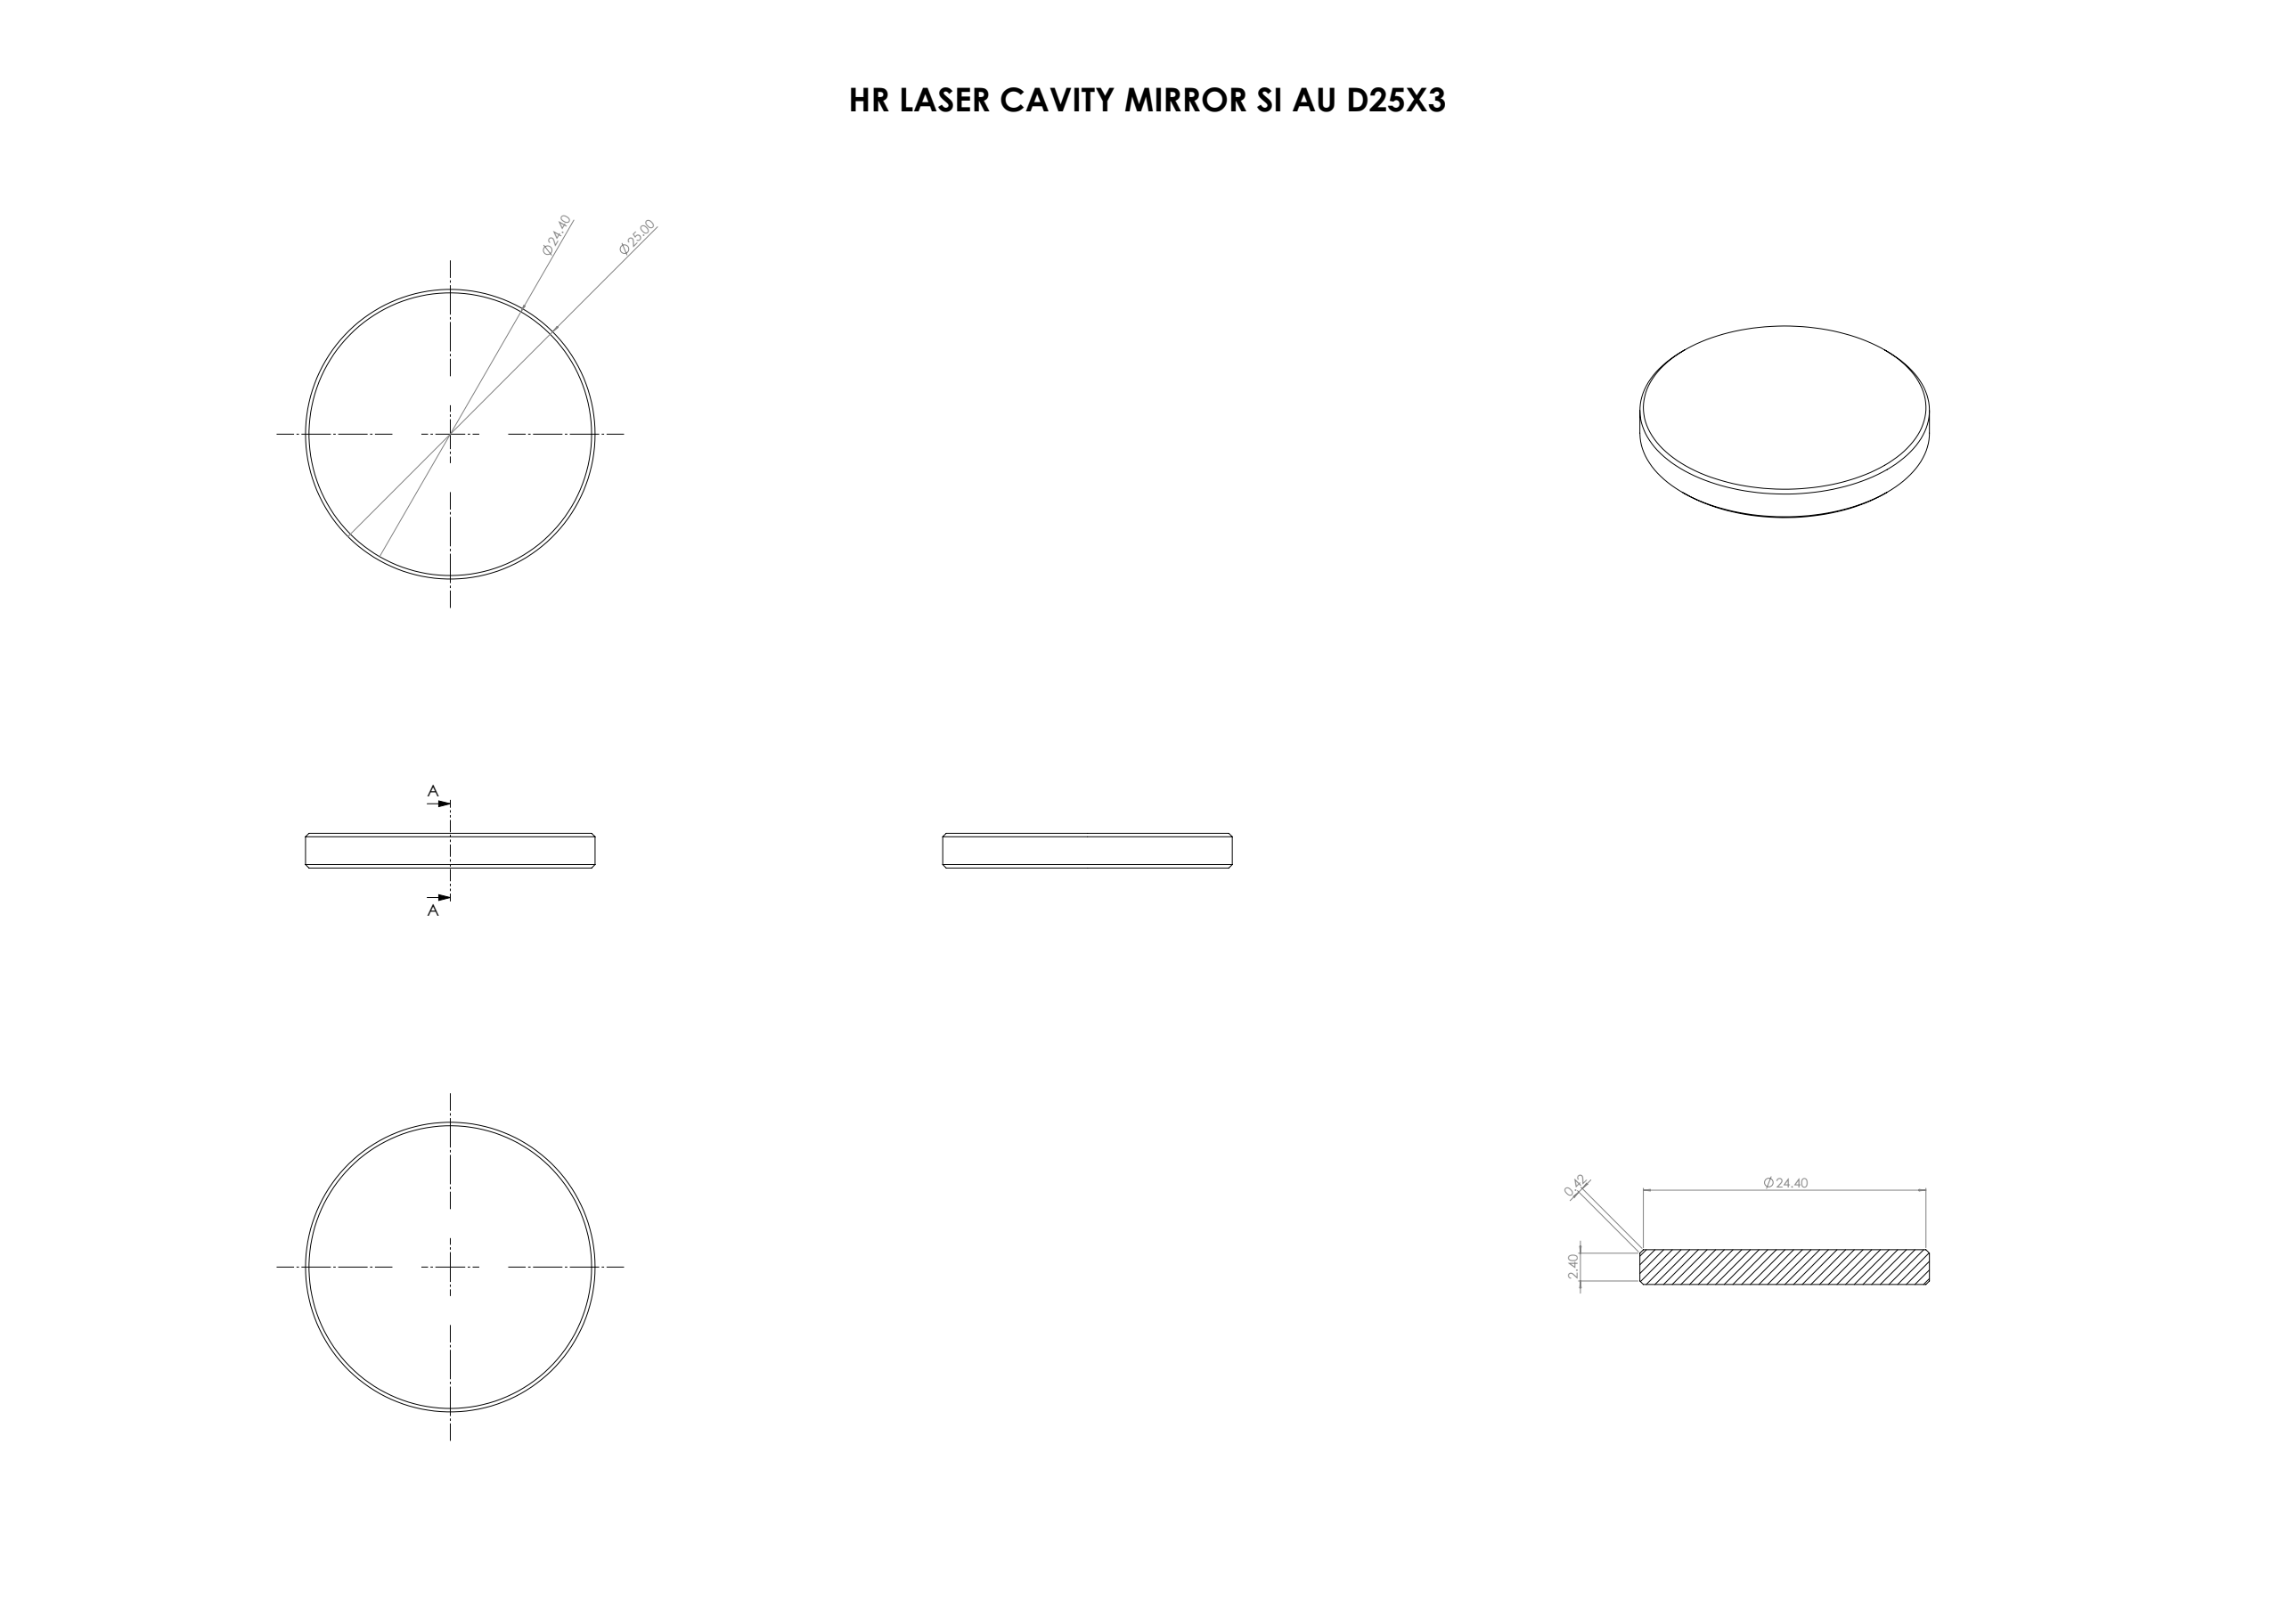
ISO-10303-21;
HEADER;
/* Generated by software containing ST-Developer
 * from STEP Tools, Inc. (www.steptools.com) 
 */

FILE_DESCRIPTION(
/* description */ (''),
/* implementation_level */ '2;1');

FILE_NAME(
/* name */ 
'06_HR_Laser_Cavity_Mirror_Si_Au_D25x3.step',
/* time_stamp */ '2026-10-20T10:06:23-07:00',
/* author */ (''),
/* organization */ (''),
/* preprocessor_version */ 'ST-DEVELOPER v20.2',
/* originating_system */ 'Autodesk Translation Framework v15.15.0.0',
/* authorisation */ '');

FILE_SCHEMA (('AUTOMOTIVE_DESIGN { 1 0 10303 214 3 1 1 }'));
ENDSEC;

DATA;
#10=MECHANICAL_DESIGN_GEOMETRIC_PRESENTATION_REPRESENTATION('',(#464),#38611);
#436=SHAPE_REPRESENTATION_RELATIONSHIP('SRR','None',#38672,#450);
#450=ADVANCED_BREP_SHAPE_REPRESENTATION('',(#478),#38601);
#464=STYLED_ITEM('',(#38871),#478);
#478=MANIFOLD_SOLID_BREP('Mirror',#16238);
#906=CYLINDRICAL_SURFACE('',#16779,1.25);
#1337=CIRCLE('',#16776,1.22);
#1338=CIRCLE('',#16778,1.25);
#1339=CIRCLE('',#16780,1.25);
#1340=CIRCLE('',#16782,1.22);
#1733=CONICAL_SURFACE('',#16777,1.235,0.785398163397449);
#1734=CONICAL_SURFACE('',#16781,1.235,0.78539816339745);
#2010=FACE_OUTER_BOUND('',#2953,.T.);
#2011=FACE_OUTER_BOUND('',#2954,.T.);
#2012=FACE_OUTER_BOUND('',#2955,.T.);
#2013=FACE_OUTER_BOUND('',#2956,.T.);
#2014=FACE_OUTER_BOUND('',#2957,.T.);
#2953=EDGE_LOOP('',(#11173));
#2954=EDGE_LOOP('',(#11174,#11175,#11176,#11177));
#2955=EDGE_LOOP('',(#11178,#11179,#11180,#11181));
#2956=EDGE_LOOP('',(#11182,#11183,#11184,#11185));
#2957=EDGE_LOOP('',(#11186));
#4081=LINE('',#23395,#5305);
#4082=LINE('',#23399,#5306);
#4083=LINE('',#23403,#5307);
#5305=VECTOR('',#18984,1.235);
#5306=VECTOR('',#18989,1.25);
#5307=VECTOR('',#18994,1.235);
#6459=VERTEX_POINT('',#23390);
#6460=VERTEX_POINT('',#23393);
#6461=VERTEX_POINT('',#23397);
#6462=VERTEX_POINT('',#23401);
#8202=EDGE_CURVE('',#6459,#6459,#1337,.T.);
#8203=EDGE_CURVE('',#6460,#6460,#1338,.T.);
#8204=EDGE_CURVE('',#6460,#6459,#4081,.T.);
#8205=EDGE_CURVE('',#6461,#6461,#1339,.T.);
#8206=EDGE_CURVE('',#6461,#6460,#4082,.T.);
#8207=EDGE_CURVE('',#6462,#6462,#1340,.T.);
#8208=EDGE_CURVE('',#6462,#6461,#4083,.T.);
#11173=ORIENTED_EDGE('',*,*,#8202,.F.);
#11174=ORIENTED_EDGE('',*,*,#8203,.F.);
#11175=ORIENTED_EDGE('',*,*,#8204,.T.);
#11176=ORIENTED_EDGE('',*,*,#8202,.T.);
#11177=ORIENTED_EDGE('',*,*,#8204,.F.);
#11178=ORIENTED_EDGE('',*,*,#8205,.F.);
#11179=ORIENTED_EDGE('',*,*,#8206,.T.);
#11180=ORIENTED_EDGE('',*,*,#8203,.T.);
#11181=ORIENTED_EDGE('',*,*,#8206,.F.);
#11182=ORIENTED_EDGE('',*,*,#8207,.F.);
#11183=ORIENTED_EDGE('',*,*,#8208,.T.);
#11184=ORIENTED_EDGE('',*,*,#8205,.T.);
#11185=ORIENTED_EDGE('',*,*,#8208,.F.);
#11186=ORIENTED_EDGE('',*,*,#8207,.T.);
#14950=PLANE('',#16775);
#14951=PLANE('',#16783);
#15553=ADVANCED_FACE('',(#2010),#14950,.T.);
#15554=ADVANCED_FACE('',(#2011),#1733,.T.);
#15555=ADVANCED_FACE('',(#2012),#906,.T.);
#15556=ADVANCED_FACE('',(#2013),#1734,.T.);
#15557=ADVANCED_FACE('',(#2014),#14951,.T.);
#16238=CLOSED_SHELL('',(#15553,#15554,#15555,#15556,#15557));
#16774=AXIS2_PLACEMENT_3D('',#23388,#18974,#18975);
#16775=AXIS2_PLACEMENT_3D('',#23389,#18976,#18977);
#16776=AXIS2_PLACEMENT_3D('',#23391,#18978,#18979);
#16777=AXIS2_PLACEMENT_3D('',#23392,#18980,#18981);
#16778=AXIS2_PLACEMENT_3D('',#23394,#18982,#18983);
#16779=AXIS2_PLACEMENT_3D('',#23396,#18985,#18986);
#16780=AXIS2_PLACEMENT_3D('',#23398,#18987,#18988);
#16781=AXIS2_PLACEMENT_3D('',#23400,#18990,#18991);
#16782=AXIS2_PLACEMENT_3D('',#23402,#18992,#18993);
#16783=AXIS2_PLACEMENT_3D('',#23404,#18995,#18996);
#18974=DIRECTION('axis',(0.,0.,1.));
#18975=DIRECTION('refdir',(1.,0.,0.));
#18976=DIRECTION('center_axis',(0.,1.,0.));
#18977=DIRECTION('ref_axis',(0.,0.,1.));
#18978=DIRECTION('center_axis',(0.,-1.,0.));
#18979=DIRECTION('ref_axis',(1.,0.,0.));
#18980=DIRECTION('center_axis',(0.,-1.,0.));
#18981=DIRECTION('ref_axis',(1.,0.,0.));
#18982=DIRECTION('center_axis',(0.,-1.,0.));
#18983=DIRECTION('ref_axis',(1.,0.,0.));
#18984=DIRECTION('',(0.707106781186548,0.707106781186547,8.65956056235494E-17));
#18985=DIRECTION('center_axis',(0.,-1.,0.));
#18986=DIRECTION('ref_axis',(1.,0.,0.));
#18987=DIRECTION('center_axis',(0.,-1.,0.));
#18988=DIRECTION('ref_axis',(1.,0.,0.));
#18989=DIRECTION('',(0.,1.,0.));
#18990=DIRECTION('center_axis',(0.,1.,0.));
#18991=DIRECTION('ref_axis',(1.,0.,0.));
#18992=DIRECTION('center_axis',(0.,-1.,0.));
#18993=DIRECTION('ref_axis',(1.,0.,0.));
#18994=DIRECTION('',(-0.707106781186549,0.707106781186546,-8.65956056235495E-17));
#18995=DIRECTION('center_axis',(0.,-1.,0.));
#18996=DIRECTION('ref_axis',(0.,0.,-1.));
#23388=CARTESIAN_POINT('',(0.,0.,0.));
#23389=CARTESIAN_POINT('Origin',(0.82,-0.4,9.7));
#23390=CARTESIAN_POINT('',(-1.62,-0.4,9.7));
#23391=CARTESIAN_POINT('Origin',(-0.4,-0.4,9.7));
#23392=CARTESIAN_POINT('Origin',(-0.4,-0.415,9.7));
#23393=CARTESIAN_POINT('',(-1.65,-0.43,9.7));
#23394=CARTESIAN_POINT('Origin',(-0.4,-0.43,9.7));
#23395=CARTESIAN_POINT('',(-1.635,-0.415,9.7));
#23396=CARTESIAN_POINT('Origin',(-0.4,-0.55,9.7));
#23397=CARTESIAN_POINT('',(-1.65,-0.67,9.7));
#23398=CARTESIAN_POINT('Origin',(-0.4,-0.67,9.7));
#23399=CARTESIAN_POINT('',(-1.65,-0.55,9.7));
#23400=CARTESIAN_POINT('Origin',(-0.4,-0.685,9.7));
#23401=CARTESIAN_POINT('',(-1.62,-0.7,9.7));
#23402=CARTESIAN_POINT('Origin',(-0.4,-0.7,9.7));
#23403=CARTESIAN_POINT('',(-1.635,-0.685,9.7));
#23404=CARTESIAN_POINT('Origin',(-0.4,-0.7,9.7));
#38585=UNCERTAINTY_MEASURE_WITH_UNIT(LENGTH_MEASURE(0.001),#38612,
'DISTANCE_ACCURACY_VALUE',
'Maximum model space distance between geometric entities at asserted c
onnectivities');
#38595=UNCERTAINTY_MEASURE_WITH_UNIT(LENGTH_MEASURE(0.001),#38612,
'DISTANCE_ACCURACY_VALUE',
'Maximum model space distance between geometric entities at asserted c
onnectivities');
#38601=(
GEOMETRIC_REPRESENTATION_CONTEXT(3)
GLOBAL_UNCERTAINTY_ASSIGNED_CONTEXT((#38585))
GLOBAL_UNIT_ASSIGNED_CONTEXT((#38612,#38614,#38615))
REPRESENTATION_CONTEXT('','3D')
);
#38611=(
GEOMETRIC_REPRESENTATION_CONTEXT(3)
GLOBAL_UNCERTAINTY_ASSIGNED_CONTEXT((#38595))
GLOBAL_UNIT_ASSIGNED_CONTEXT((#38612,#38614,#38615))
REPRESENTATION_CONTEXT('','3D')
);
#38612=(
LENGTH_UNIT()
NAMED_UNIT(*)
SI_UNIT(.CENTI.,.METRE.)
);
#38614=(
NAMED_UNIT(*)
PLANE_ANGLE_UNIT()
SI_UNIT($,.RADIAN.)
);
#38615=(
NAMED_UNIT(*)
SI_UNIT($,.STERADIAN.)
SOLID_ANGLE_UNIT()
);
#38621=SHAPE_DEFINITION_REPRESENTATION(#38636,#38672);
#38636=PRODUCT_DEFINITION_SHAPE('',$,#38688);
#38672=SHAPE_REPRESENTATION('',(#16774),#38601);
#38682=PRODUCT_DEFINITION_CONTEXT('part definition',#38729,'design');
#38688=PRODUCT_DEFINITION('2026-10-19-02-31-35-057',
'06_HR_Laser_Cavity_Mirror_Si_Au_D25x3',#38703,#38682);
#38703=PRODUCT_DEFINITION_FORMATION('',$,#38736);
#38729=APPLICATION_CONTEXT(
'Core Data for Automotive Mechanical Design Process');
#38730=PRODUCT_CONTEXT('part definition',#38729,'mechanical');
#38736=PRODUCT('2026-10-19-02-31-35-057',
'06_HR_Laser_Cavity_Mirror_Si_Au_D25x3',$,(#38730));
#38865=COLOUR_RGB('Sky Blue',0.24,0.69,0.87);
#38866=FILL_AREA_STYLE_COLOUR('',#38865);
#38867=FILL_AREA_STYLE('',(#38866));
#38868=SURFACE_STYLE_FILL_AREA(#38867);
#38869=SURFACE_SIDE_STYLE('',(#38868));
#38870=SURFACE_STYLE_USAGE(.BOTH.,#38869);
#38871=PRESENTATION_STYLE_ASSIGNMENT((#38870));
ENDSEC;
END-ISO-10303-21;
